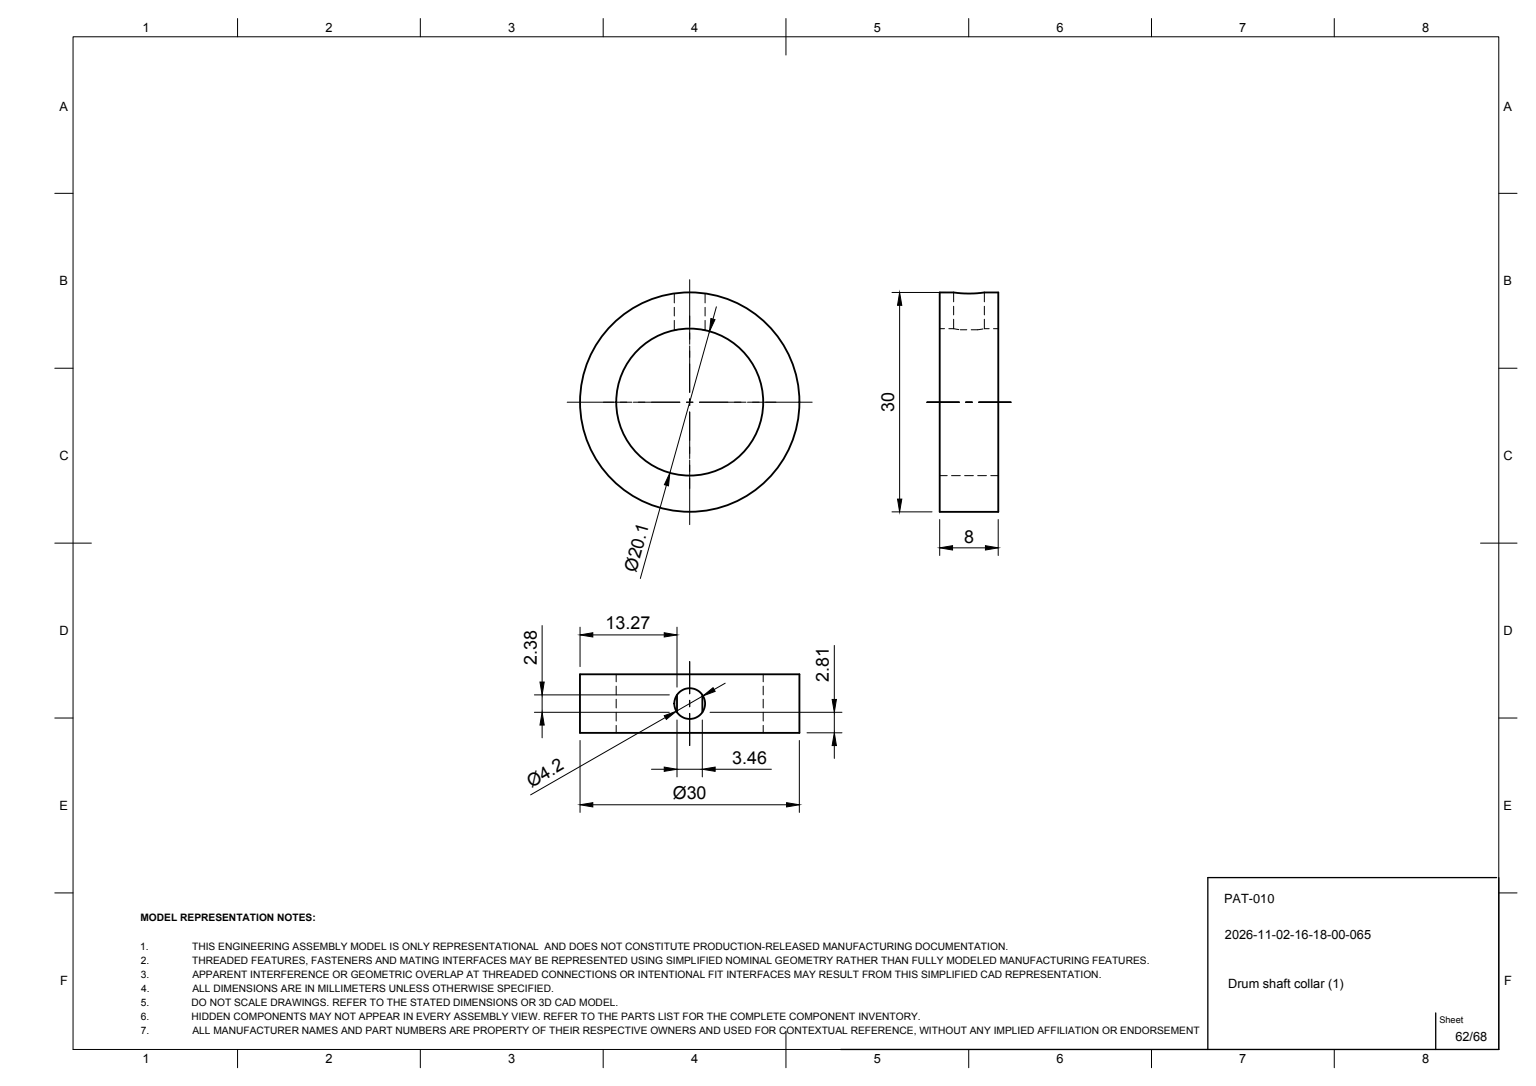
ISO-10303-21;
HEADER;
/* Generated by software containing ST-Developer
 * from STEP Tools, Inc. (www.steptools.com) 
 */

FILE_DESCRIPTION(
/* description */ ('Belt conveyor head drive unit'),
/* implementation_level */ '2;1');

FILE_NAME(
/* name */ 'Drum shaft collar (1).step',
/* time_stamp */ '2026-10-28T03:26:19-07:00',
/* author */ (''),
/* organization */ (''),
/* preprocessor_version */ 'ST-DEVELOPER v20.2',
/* originating_system */ 'Autodesk Translation Framework v15.17.0.0',
/* authorisation */ '');

FILE_SCHEMA (('AUTOMOTIVE_DESIGN { 1 0 10303 214 3 1 1 }'));
ENDSEC;

DATA;
#10=MECHANICAL_DESIGN_GEOMETRIC_PRESENTATION_REPRESENTATION('',(#923),#27069);
#611=B_SPLINE_CURVE_WITH_KNOTS('',3,(#25515,#25516,#25517,#25518,#25519,
#25520,#25521,#25522,#25523,#25524,#25525,#25526,#25527,#25528),
 .UNSPECIFIED.,.F.,.F.,(4,2,2,2,2,2,4),(0.756005737987017,0.793568827564644,
0.872922520054199,0.952276212543754,1.03162990503331,1.11098359752286,1.14854668710049),
 .UNSPECIFIED.);
#612=B_SPLINE_CURVE_WITH_KNOTS('',3,(#25534,#25535,#25536,#25537,#25538,
#25539,#25540,#25541,#25542,#25543,#25544,#25545,#25546,#25547,#25548,#25549,
#25550,#25551),.UNSPECIFIED.,.F.,.F.,(4,2,2,2,2,2,2,2,4),(0.,0.0792165807733624,
0.158433161546725,0.237648697074569,0.316864232602414,0.396079768130259,
0.475295303658103,0.554511884431465,0.633728465204828),.UNSPECIFIED.);
#613=B_SPLINE_CURVE_WITH_KNOTS('',3,(#25552,#25553,#25554,#25555,#25556,
#25557,#25558,#25559,#25560,#25561,#25562,#25563,#25564,#25565,#25566,#25567,
#25568,#25569),.UNSPECIFIED.,.F.,.F.,(4,2,2,2,2,2,2,2,4),(0.633728465204828,
0.71294504597819,0.792161626751553,0.871377162279397,0.950592697807242,
1.02980823333509,1.10902376886293,1.18824034963629,1.26745693040966),
 .UNSPECIFIED.);
#614=B_SPLINE_CURVE_WITH_KNOTS('',3,(#25572,#25573,#25574,#25575,#25576,
#25577,#25578,#25579,#25580,#25581,#25582,#25583,#25584,#25585),
 .UNSPECIFIED.,.F.,.F.,(4,2,2,2,2,2,4),(0.121154929624508,0.158718019202141,
0.238071711691696,0.317425404181251,0.396779096670806,0.476132789160361,
0.513695878737978),.UNSPECIFIED.);
#769=SHAPE_REPRESENTATION_RELATIONSHIP('SRR','None',#27418,#838);
#838=ADVANCED_BREP_SHAPE_REPRESENTATION('',(#1004),#27060);
#923=STYLED_ITEM('',(#27797),#1004);
#1004=MANIFOLD_SOLID_BREP('Body1',#13792);
#1246=FACE_BOUND('',#3316,.T.);
#1247=FACE_BOUND('',#3318,.T.);
#1248=FACE_BOUND('',#3320,.T.);
#1249=FACE_BOUND('',#3322,.T.);
#1590=PLANE('',#15945);
#1591=PLANE('',#15950);
#1592=PLANE('',#15957);
#1593=PLANE('',#15958);
#2278=FACE_OUTER_BOUND('',#3312,.T.);
#2279=FACE_OUTER_BOUND('',#3313,.T.);
#2280=FACE_OUTER_BOUND('',#3314,.T.);
#2281=FACE_OUTER_BOUND('',#3315,.T.);
#2282=FACE_OUTER_BOUND('',#3317,.T.);
#2283=FACE_OUTER_BOUND('',#3319,.T.);
#2284=FACE_OUTER_BOUND('',#3321,.T.);
#3312=EDGE_LOOP('',(#11726,#11727));
#3313=EDGE_LOOP('',(#11728,#11729,#11730,#11731,#11732,#11733,#11734,#11735,
#11736));
#3314=EDGE_LOOP('',(#11737,#11738,#11739));
#3315=EDGE_LOOP('',(#11740,#11741,#11742,#11743));
#3316=EDGE_LOOP('',(#11744,#11745,#11746,#11747));
#3317=EDGE_LOOP('',(#11748,#11749,#11750,#11751));
#3318=EDGE_LOOP('',(#11752,#11753));
#3319=EDGE_LOOP('',(#11754));
#3320=EDGE_LOOP('',(#11755));
#3321=EDGE_LOOP('',(#11756));
#3322=EDGE_LOOP('',(#11757));
#4134=LINE('',#25511,#4926);
#4135=LINE('',#25532,#4927);
#4136=LINE('',#25587,#4928);
#4137=LINE('',#25592,#4929);
#4138=LINE('',#25598,#4930);
#4926=VECTOR('',#19838,1.);
#4927=VECTOR('',#19845,0.21);
#4928=VECTOR('',#19850,1.);
#4929=VECTOR('',#19855,1.005);
#4930=VECTOR('',#19862,1.5);
#5740=CIRCLE('',#15946,0.21);
#5741=CIRCLE('',#15948,0.21);
#5742=CIRCLE('',#15949,0.21);
#5743=CIRCLE('',#15952,1.005);
#5744=CIRCLE('',#15953,1.005);
#5745=CIRCLE('',#15955,1.5);
#5746=CIRCLE('',#15956,1.5);
#6900=VERTEX_POINT('',#25509);
#6901=VERTEX_POINT('',#25510);
#6902=VERTEX_POINT('',#25514);
#6903=VERTEX_POINT('',#25529);
#6904=VERTEX_POINT('',#25531);
#6905=VERTEX_POINT('',#25533);
#6906=VERTEX_POINT('',#25570);
#6907=VERTEX_POINT('',#25589);
#6908=VERTEX_POINT('',#25591);
#6909=VERTEX_POINT('',#25595);
#6910=VERTEX_POINT('',#25597);
#8555=EDGE_CURVE('',#6900,#6901,#4134,.T.);
#8556=EDGE_CURVE('',#6900,#6901,#5740,.T.);
#8557=EDGE_CURVE('',#6902,#6900,#611,.T.);
#8558=EDGE_CURVE('',#6903,#6902,#5741,.T.);
#8559=EDGE_CURVE('',#6903,#6904,#4135,.T.);
#8560=EDGE_CURVE('',#6905,#6904,#612,.T.);
#8561=EDGE_CURVE('',#6904,#6905,#613,.T.);
#8562=EDGE_CURVE('',#6906,#6903,#5742,.T.);
#8563=EDGE_CURVE('',#6901,#6906,#614,.T.);
#8564=EDGE_CURVE('',#6906,#6902,#4136,.T.);
#8565=EDGE_CURVE('',#6907,#6907,#5743,.T.);
#8566=EDGE_CURVE('',#6907,#6908,#4137,.T.);
#8567=EDGE_CURVE('',#6908,#6908,#5744,.T.);
#8568=EDGE_CURVE('',#6909,#6909,#5745,.T.);
#8569=EDGE_CURVE('',#6909,#6910,#4138,.T.);
#8570=EDGE_CURVE('',#6910,#6910,#5746,.T.);
#11726=ORIENTED_EDGE('',*,*,#8555,.F.);
#11727=ORIENTED_EDGE('',*,*,#8556,.T.);
#11728=ORIENTED_EDGE('',*,*,#8557,.F.);
#11729=ORIENTED_EDGE('',*,*,#8558,.F.);
#11730=ORIENTED_EDGE('',*,*,#8559,.T.);
#11731=ORIENTED_EDGE('',*,*,#8560,.F.);
#11732=ORIENTED_EDGE('',*,*,#8561,.F.);
#11733=ORIENTED_EDGE('',*,*,#8559,.F.);
#11734=ORIENTED_EDGE('',*,*,#8562,.F.);
#11735=ORIENTED_EDGE('',*,*,#8563,.F.);
#11736=ORIENTED_EDGE('',*,*,#8556,.F.);
#11737=ORIENTED_EDGE('',*,*,#8564,.F.);
#11738=ORIENTED_EDGE('',*,*,#8562,.T.);
#11739=ORIENTED_EDGE('',*,*,#8558,.T.);
#11740=ORIENTED_EDGE('',*,*,#8565,.F.);
#11741=ORIENTED_EDGE('',*,*,#8566,.T.);
#11742=ORIENTED_EDGE('',*,*,#8567,.T.);
#11743=ORIENTED_EDGE('',*,*,#8566,.F.);
#11744=ORIENTED_EDGE('',*,*,#8563,.T.);
#11745=ORIENTED_EDGE('',*,*,#8564,.T.);
#11746=ORIENTED_EDGE('',*,*,#8557,.T.);
#11747=ORIENTED_EDGE('',*,*,#8555,.T.);
#11748=ORIENTED_EDGE('',*,*,#8568,.F.);
#11749=ORIENTED_EDGE('',*,*,#8569,.T.);
#11750=ORIENTED_EDGE('',*,*,#8570,.T.);
#11751=ORIENTED_EDGE('',*,*,#8569,.F.);
#11752=ORIENTED_EDGE('',*,*,#8560,.T.);
#11753=ORIENTED_EDGE('',*,*,#8561,.T.);
#11754=ORIENTED_EDGE('',*,*,#8568,.T.);
#11755=ORIENTED_EDGE('',*,*,#8565,.T.);
#11756=ORIENTED_EDGE('',*,*,#8570,.F.);
#11757=ORIENTED_EDGE('',*,*,#8567,.F.);
#12806=CYLINDRICAL_SURFACE('',#15947,0.21);
#12807=CYLINDRICAL_SURFACE('',#15951,1.005);
#12808=CYLINDRICAL_SURFACE('',#15954,1.5);
#13557=ADVANCED_FACE('',(#2278),#1590,.T.);
#13558=ADVANCED_FACE('',(#2279),#12806,.F.);
#13559=ADVANCED_FACE('',(#2280),#1591,.T.);
#13560=ADVANCED_FACE('',(#2281,#1246),#12807,.F.);
#13561=ADVANCED_FACE('',(#2282,#1247),#12808,.T.);
#13562=ADVANCED_FACE('',(#2283,#1248),#1592,.T.);
#13563=ADVANCED_FACE('',(#2284,#1249),#1593,.F.);
#13792=CLOSED_SHELL('',(#13557,#13558,#13559,#13560,#13561,#13562,#13563));
#15944=AXIS2_PLACEMENT_3D('',#25507,#19834,#19835);
#15945=AXIS2_PLACEMENT_3D('',#25508,#19836,#19837);
#15946=AXIS2_PLACEMENT_3D('',#25512,#19839,#19840);
#15947=AXIS2_PLACEMENT_3D('',#25513,#19841,#19842);
#15948=AXIS2_PLACEMENT_3D('',#25530,#19843,#19844);
#15949=AXIS2_PLACEMENT_3D('',#25571,#19846,#19847);
#15950=AXIS2_PLACEMENT_3D('',#25586,#19848,#19849);
#15951=AXIS2_PLACEMENT_3D('',#25588,#19851,#19852);
#15952=AXIS2_PLACEMENT_3D('',#25590,#19853,#19854);
#15953=AXIS2_PLACEMENT_3D('',#25593,#19856,#19857);
#15954=AXIS2_PLACEMENT_3D('',#25594,#19858,#19859);
#15955=AXIS2_PLACEMENT_3D('',#25596,#19860,#19861);
#15956=AXIS2_PLACEMENT_3D('',#25599,#19863,#19864);
#15957=AXIS2_PLACEMENT_3D('',#25600,#19865,#19866);
#15958=AXIS2_PLACEMENT_3D('',#25601,#19867,#19868);
#19834=DIRECTION('axis',(0.,0.,1.));
#19835=DIRECTION('refdir',(1.,0.,0.));
#19836=DIRECTION('center_axis',(0.,0.,1.));
#19837=DIRECTION('ref_axis',(1.,0.,0.));
#19838=DIRECTION('',(0.,1.,0.));
#19839=DIRECTION('center_axis',(0.,0.,1.));
#19840=DIRECTION('ref_axis',(1.,0.,0.));
#19841=DIRECTION('center_axis',(0.,0.,1.));
#19842=DIRECTION('ref_axis',(1.,0.,0.));
#19843=DIRECTION('center_axis',(0.,0.,1.));
#19844=DIRECTION('ref_axis',(1.,0.,0.));
#19845=DIRECTION('',(0.,0.,1.));
#19846=DIRECTION('center_axis',(0.,0.,1.));
#19847=DIRECTION('ref_axis',(1.,0.,0.));
#19848=DIRECTION('center_axis',(0.,0.,1.));
#19849=DIRECTION('ref_axis',(1.,0.,0.));
#19850=DIRECTION('',(0.,-1.,0.));
#19851=DIRECTION('center_axis',(0.,1.,0.));
#19852=DIRECTION('ref_axis',(1.,0.,0.));
#19853=DIRECTION('center_axis',(0.,-1.,0.));
#19854=DIRECTION('ref_axis',(1.,0.,0.));
#19855=DIRECTION('',(0.,-1.,0.));
#19856=DIRECTION('center_axis',(0.,-1.,0.));
#19857=DIRECTION('ref_axis',(1.,0.,0.));
#19858=DIRECTION('center_axis',(0.,1.,0.));
#19859=DIRECTION('ref_axis',(1.,0.,0.));
#19860=DIRECTION('center_axis',(0.,1.,0.));
#19861=DIRECTION('ref_axis',(1.,0.,0.));
#19862=DIRECTION('',(0.,-1.,0.));
#19863=DIRECTION('center_axis',(0.,1.,0.));
#19864=DIRECTION('ref_axis',(1.,0.,0.));
#19865=DIRECTION('center_axis',(0.,1.,0.));
#19866=DIRECTION('ref_axis',(1.,0.,0.));
#19867=DIRECTION('center_axis',(0.,1.,0.));
#19868=DIRECTION('ref_axis',(1.,0.,0.));
#25507=CARTESIAN_POINT('',(0.,0.,0.));
#25508=CARTESIAN_POINT('Origin',(6.97091003018116,42.85,7.99));
#25509=CARTESIAN_POINT('',(7.14389846910121,42.7309411910021,7.99));
#25510=CARTESIAN_POINT('',(7.14389846910121,42.9690588089979,7.99));
#25511=CARTESIAN_POINT('',(7.14389846910121,42.45,7.99));
#25512=CARTESIAN_POINT('Origin',(6.97091003018116,42.85,7.99));
#25513=CARTESIAN_POINT('Origin',(6.97091003018116,42.85,7.99));
#25514=CARTESIAN_POINT('',(6.7979215912611,42.7309411910021,7.99));
#25515=CARTESIAN_POINT('Ctrl Pts',(6.7979215912611,42.7309411910021,7.99));
#25516=CARTESIAN_POINT('Ctrl Pts',(6.80531516486984,42.7201985776047,7.99129192197638));
#25517=CARTESIAN_POINT('Ctrl Pts',(6.81361289145555,42.7103122906273,7.99265394943905));
#25518=CARTESIAN_POINT('Ctrl Pts',(6.84101795633608,42.6829072257467,7.9967480843909));
#25519=CARTESIAN_POINT('Ctrl Pts',(6.86457986242187,42.6667579436671,7.99969589327637));
#25520=CARTESIAN_POINT('Ctrl Pts',(6.91629712554875,42.6453022060351,8.00385029472357));
#25521=CARTESIAN_POINT('Ctrl Pts',(6.9444587993513,42.64,8.005));
#25522=CARTESIAN_POINT('Ctrl Pts',(6.99736126101101,42.64,8.005));
#25523=CARTESIAN_POINT('Ctrl Pts',(7.02552293481356,42.6453022060351,8.00385029472357));
#25524=CARTESIAN_POINT('Ctrl Pts',(7.07724019794044,42.6667579436671,7.99969589327638));
#25525=CARTESIAN_POINT('Ctrl Pts',(7.10080210402623,42.6829072257467,7.9967480843909));
#25526=CARTESIAN_POINT('Ctrl Pts',(7.12820716890676,42.7103122906273,7.99265394943905));
#25527=CARTESIAN_POINT('Ctrl Pts',(7.13650489549247,42.7201985776047,7.99129192197638));
#25528=CARTESIAN_POINT('Ctrl Pts',(7.14389846910121,42.7309411910021,7.99));
#25529=CARTESIAN_POINT('',(6.76091003018116,42.85,7.99));
#25530=CARTESIAN_POINT('Origin',(6.97091003018116,42.85,7.99));
#25531=CARTESIAN_POINT('',(6.76091003018116,42.85,8.48522725533839));
#25532=CARTESIAN_POINT('',(6.76091003018116,42.85,7.99));
#25533=CARTESIAN_POINT('',(7.18091003018116,42.85,8.48522725533839));
#25534=CARTESIAN_POINT('Ctrl Pts',(7.18091003018116,42.85,8.48522725533839));
#25535=CARTESIAN_POINT('Ctrl Pts',(7.18091003018116,42.8235944730755,8.48522725533839));
#25536=CARTESIAN_POINT('Ctrl Pts',(7.17562576745075,42.7954529259093,8.48600415954412));
#25537=CARTESIAN_POINT('Ctrl Pts',(7.15418379321749,42.7437237310949,8.48880073282317));
#25538=CARTESIAN_POINT('Ctrl Pts',(7.13802795415155,42.720133075872,8.49077897157582));
#25539=CARTESIAN_POINT('Ctrl Pts',(7.10077720006852,42.682882321789,8.49448481141327));
#25540=CARTESIAN_POINT('Ctrl Pts',(7.07718643848692,42.6667262899986,8.49645455657129));
#25541=CARTESIAN_POINT('Ctrl Pts',(7.02545688158705,42.6452841751738,8.49923165515646));
#25542=CARTESIAN_POINT('Ctrl Pts',(6.99731520869044,42.64,8.5));
#25543=CARTESIAN_POINT('Ctrl Pts',(6.94450485167187,42.64,8.5));
#25544=CARTESIAN_POINT('Ctrl Pts',(6.91636317877526,42.6452841751738,8.49923165515646));
#25545=CARTESIAN_POINT('Ctrl Pts',(6.86463362187539,42.6667262899986,8.49645455657129));
#25546=CARTESIAN_POINT('Ctrl Pts',(6.84104286029379,42.682882321789,8.49448481141327));
#25547=CARTESIAN_POINT('Ctrl Pts',(6.80379210621076,42.720133075872,8.49077897157582));
#25548=CARTESIAN_POINT('Ctrl Pts',(6.78763626714482,42.7437237310949,8.48880073282317));
#25549=CARTESIAN_POINT('Ctrl Pts',(6.76619429291156,42.7954529259093,8.48600415954412));
#25550=CARTESIAN_POINT('Ctrl Pts',(6.76091003018116,42.8235944730756,8.48522725533839));
#25551=CARTESIAN_POINT('Ctrl Pts',(6.76091003018116,42.85,8.48522725533839));
#25552=CARTESIAN_POINT('Ctrl Pts',(6.76091003018116,42.85,8.48522725533839));
#25553=CARTESIAN_POINT('Ctrl Pts',(6.76091003018116,42.8764055269245,8.48522725533839));
#25554=CARTESIAN_POINT('Ctrl Pts',(6.76619429291156,42.9045470740907,8.48600415954412));
#25555=CARTESIAN_POINT('Ctrl Pts',(6.78763626714482,42.9562762689051,8.48880073282317));
#25556=CARTESIAN_POINT('Ctrl Pts',(6.80379210621076,42.979866924128,8.49077897157582));
#25557=CARTESIAN_POINT('Ctrl Pts',(6.84104286029379,43.017117678211,8.49448481141327));
#25558=CARTESIAN_POINT('Ctrl Pts',(6.86463362187539,43.0332737100014,8.49645455657129));
#25559=CARTESIAN_POINT('Ctrl Pts',(6.91636317877526,43.0547158248262,8.49923165515646));
#25560=CARTESIAN_POINT('Ctrl Pts',(6.94450485167187,43.06,8.5));
#25561=CARTESIAN_POINT('Ctrl Pts',(6.99731520869044,43.06,8.5));
#25562=CARTESIAN_POINT('Ctrl Pts',(7.02545688158705,43.0547158248262,8.49923165515646));
#25563=CARTESIAN_POINT('Ctrl Pts',(7.07718643848692,43.0332737100014,8.49645455657129));
#25564=CARTESIAN_POINT('Ctrl Pts',(7.10077720006852,43.017117678211,8.49448481141327));
#25565=CARTESIAN_POINT('Ctrl Pts',(7.13802795415155,42.979866924128,8.49077897157582));
#25566=CARTESIAN_POINT('Ctrl Pts',(7.15418379321749,42.9562762689051,8.48880073282317));
#25567=CARTESIAN_POINT('Ctrl Pts',(7.17562576745075,42.9045470740907,8.48600415954412));
#25568=CARTESIAN_POINT('Ctrl Pts',(7.18091003018116,42.8764055269245,8.48522725533839));
#25569=CARTESIAN_POINT('Ctrl Pts',(7.18091003018116,42.85,8.48522725533839));
#25570=CARTESIAN_POINT('',(6.7979215912611,42.9690588089979,7.99));
#25571=CARTESIAN_POINT('Origin',(6.97091003018116,42.85,7.99));
#25572=CARTESIAN_POINT('Ctrl Pts',(7.14389846910122,42.9690588089979,7.99));
#25573=CARTESIAN_POINT('Ctrl Pts',(7.13650489549248,42.9798014223953,7.99129192197638));
#25574=CARTESIAN_POINT('Ctrl Pts',(7.12820716890676,42.9896877093727,7.99265394943905));
#25575=CARTESIAN_POINT('Ctrl Pts',(7.10080210402623,43.0170927742533,7.9967480843909));
#25576=CARTESIAN_POINT('Ctrl Pts',(7.07724019794044,43.033242056333,7.99969589327637));
#25577=CARTESIAN_POINT('Ctrl Pts',(7.02552293481357,43.0546977939649,8.00385029472357));
#25578=CARTESIAN_POINT('Ctrl Pts',(6.99736126101101,43.06,8.005));
#25579=CARTESIAN_POINT('Ctrl Pts',(6.9444587993513,43.06,8.005));
#25580=CARTESIAN_POINT('Ctrl Pts',(6.91629712554875,43.0546977939649,8.00385029472357));
#25581=CARTESIAN_POINT('Ctrl Pts',(6.86457986242187,43.033242056333,7.99969589327637));
#25582=CARTESIAN_POINT('Ctrl Pts',(6.84101795633608,43.0170927742533,7.9967480843909));
#25583=CARTESIAN_POINT('Ctrl Pts',(6.81361289145555,42.9896877093727,7.99265394943905));
#25584=CARTESIAN_POINT('Ctrl Pts',(6.80531516486984,42.9798014223953,7.99129192197638));
#25585=CARTESIAN_POINT('Ctrl Pts',(6.7979215912611,42.9690588089979,7.99));
#25586=CARTESIAN_POINT('Origin',(6.97091003018116,42.85,7.99));
#25587=CARTESIAN_POINT('',(6.7979215912611,42.45,7.99));
#25588=CARTESIAN_POINT('Origin',(6.97091003018116,42.45,7.));
#25589=CARTESIAN_POINT('',(5.96591003018116,43.25,7.));
#25590=CARTESIAN_POINT('Origin',(6.97091003018116,43.25,7.));
#25591=CARTESIAN_POINT('',(5.96591003018116,42.45,7.));
#25592=CARTESIAN_POINT('',(5.96591003018116,42.45,7.));
#25593=CARTESIAN_POINT('Origin',(6.97091003018116,42.45,7.));
#25594=CARTESIAN_POINT('Origin',(6.97091003018116,42.45,7.));
#25595=CARTESIAN_POINT('',(5.47091003018116,43.25,7.));
#25596=CARTESIAN_POINT('Origin',(6.97091003018116,43.25,7.));
#25597=CARTESIAN_POINT('',(5.47091003018116,42.45,7.));
#25598=CARTESIAN_POINT('',(5.47091003018116,42.45,7.));
#25599=CARTESIAN_POINT('Origin',(6.97091003018116,42.45,7.));
#25600=CARTESIAN_POINT('Origin',(6.97091003018116,43.25,7.));
#25601=CARTESIAN_POINT('Origin',(6.97091003018116,42.45,7.));
#26983=UNCERTAINTY_MEASURE_WITH_UNIT(LENGTH_MEASURE(0.001),#27070,
'DISTANCE_ACCURACY_VALUE',
'Maximum model space distance between geometric entities at asserted c
onnectivities');
#26992=UNCERTAINTY_MEASURE_WITH_UNIT(LENGTH_MEASURE(0.001),#27070,
'DISTANCE_ACCURACY_VALUE',
'Maximum model space distance between geometric entities at asserted c
onnectivities');
#27060=(
GEOMETRIC_REPRESENTATION_CONTEXT(3)
GLOBAL_UNCERTAINTY_ASSIGNED_CONTEXT((#26983))
GLOBAL_UNIT_ASSIGNED_CONTEXT((#27070,#27072,#27073))
REPRESENTATION_CONTEXT('','3D')
);
#27069=(
GEOMETRIC_REPRESENTATION_CONTEXT(3)
GLOBAL_UNCERTAINTY_ASSIGNED_CONTEXT((#26992))
GLOBAL_UNIT_ASSIGNED_CONTEXT((#27070,#27072,#27073))
REPRESENTATION_CONTEXT('','3D')
);
#27070=(
LENGTH_UNIT()
NAMED_UNIT(*)
SI_UNIT(.CENTI.,.METRE.)
);
#27072=(
NAMED_UNIT(*)
PLANE_ANGLE_UNIT()
SI_UNIT($,.RADIAN.)
);
#27073=(
NAMED_UNIT(*)
SI_UNIT($,.STERADIAN.)
SOLID_ANGLE_UNIT()
);
#27141=SHAPE_DEFINITION_REPRESENTATION(#27229,#27418);
#27229=PRODUCT_DEFINITION_SHAPE('',$,#27495);
#27418=SHAPE_REPRESENTATION('',(#15944),#27060);
#27427=PRODUCT_DEFINITION_CONTEXT('part definition',#27657,'design');
#27495=PRODUCT_DEFINITION('Drum shaft collar (1)','Drum shaft collar (1)',
#27571,#27427);
#27571=PRODUCT_DEFINITION_FORMATION('',$,#27726);
#27657=APPLICATION_CONTEXT(
'Core Data for Automotive Mechanical Design Process');
#27658=PRODUCT_CONTEXT('part definition',#27657,'mechanical');
#27726=PRODUCT('Drum shaft collar (1)','Drum shaft collar (1)',
'Drum shaft collar (1)',(#27658));
#27791=COLOUR_RGB('Grey',0.48,0.52,0.57);
#27792=FILL_AREA_STYLE_COLOUR('',#27791);
#27793=FILL_AREA_STYLE('',(#27792));
#27794=SURFACE_STYLE_FILL_AREA(#27793);
#27795=SURFACE_SIDE_STYLE('',(#27794));
#27796=SURFACE_STYLE_USAGE(.BOTH.,#27795);
#27797=PRESENTATION_STYLE_ASSIGNMENT((#27796));
ENDSEC;
END-ISO-10303-21;
